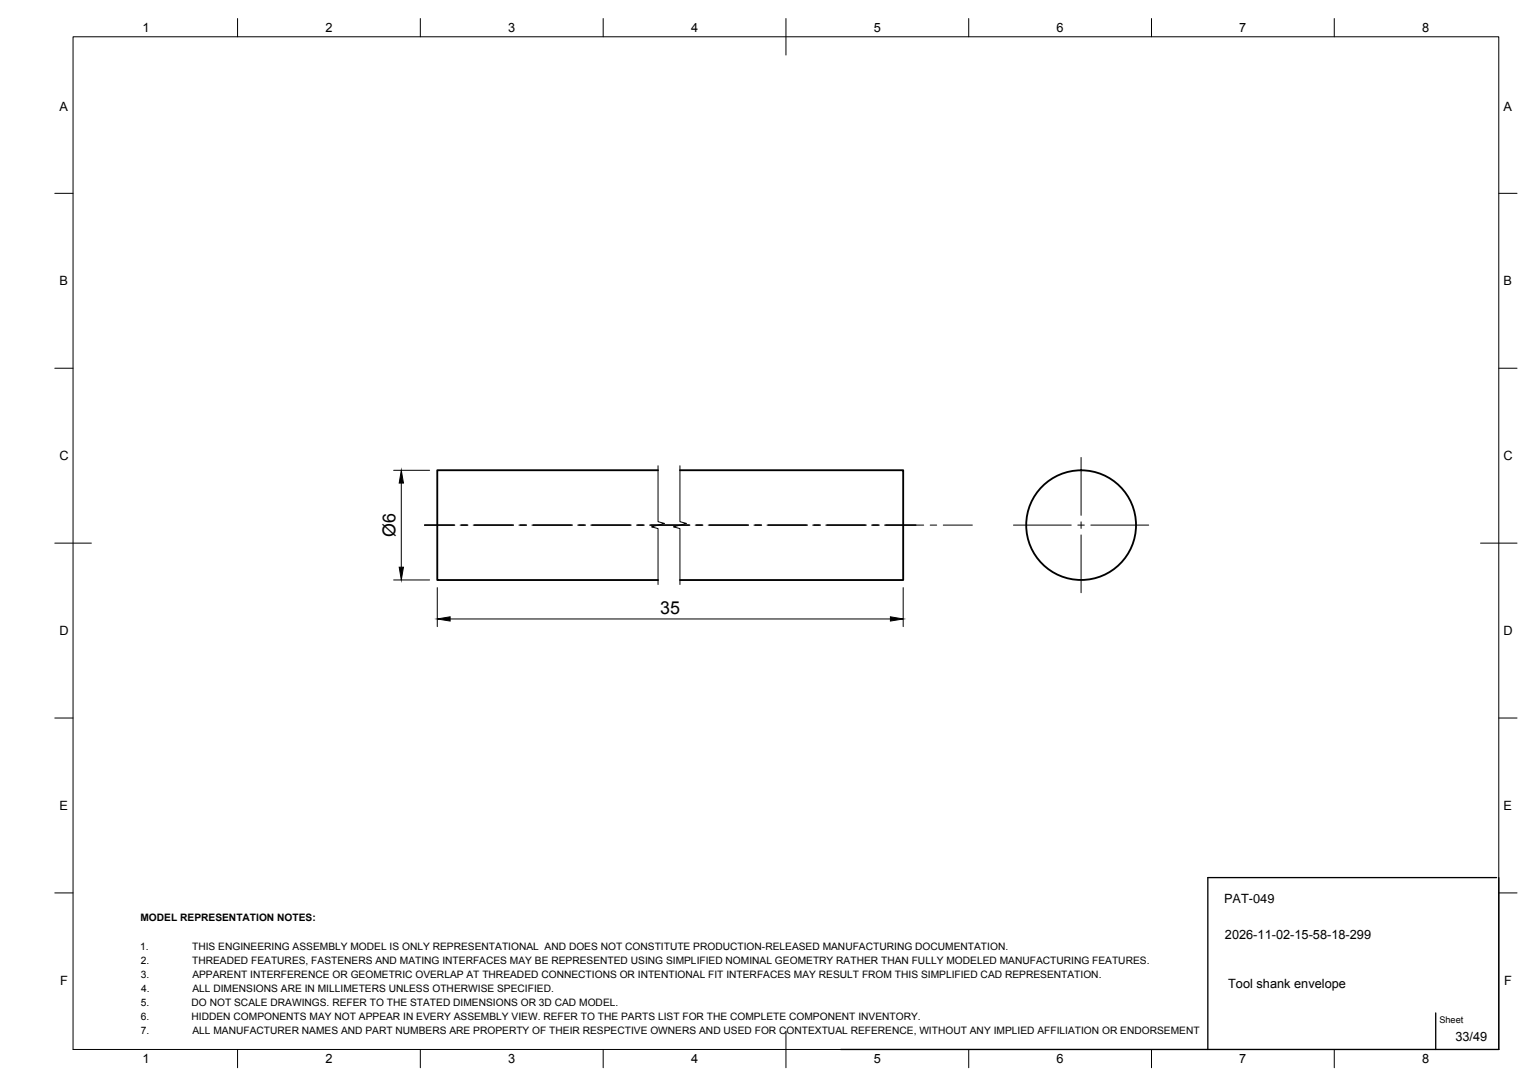
ISO-10303-21;
HEADER;
/* Generated by software containing ST-Developer
 * from STEP Tools, Inc. (www.steptools.com) 
 */

FILE_DESCRIPTION(
/* description */ ('Hand drill press frame (manual)'),
/* implementation_level */ '2;1');

FILE_NAME(
/* name */ 'Tool shank envelope.step',
/* time_stamp */ '2026-10-28T03:25:28-07:00',
/* author */ (''),
/* organization */ (''),
/* preprocessor_version */ 'ST-DEVELOPER v20.2',
/* originating_system */ 'Autodesk Translation Framework v15.17.0.0',
/* authorisation */ '');

FILE_SCHEMA (('AUTOMOTIVE_DESIGN { 1 0 10303 214 3 1 1 }'));
ENDSEC;

DATA;
#10=MECHANICAL_DESIGN_GEOMETRIC_PRESENTATION_REPRESENTATION('',(#651),#33299);
#554=SHAPE_REPRESENTATION_RELATIONSHIP('SRR','None',#33515,#599);
#599=ADVANCED_BREP_SHAPE_REPRESENTATION('',(#702),#33277);
#651=STYLED_ITEM('',(#33807),#702);
#702=MANIFOLD_SOLID_BREP('Body1',#12670);
#1219=PLANE('',#13959);
#1220=PLANE('',#13960);
#1801=FACE_OUTER_BOUND('',#2622,.T.);
#1802=FACE_OUTER_BOUND('',#2623,.T.);
#1803=FACE_OUTER_BOUND('',#2624,.T.);
#2622=EDGE_LOOP('',(#10757,#10758,#10759,#10760));
#2623=EDGE_LOOP('',(#10761));
#2624=EDGE_LOOP('',(#10762));
#3747=LINE('',#20875,#4912);
#4912=VECTOR('',#16770,0.3);
#5485=CIRCLE('',#13957,0.3);
#5486=CIRCLE('',#13958,0.3);
#6399=VERTEX_POINT('',#20872);
#6400=VERTEX_POINT('',#20874);
#7907=EDGE_CURVE('',#6399,#6399,#5485,.T.);
#7908=EDGE_CURVE('',#6399,#6400,#3747,.T.);
#7909=EDGE_CURVE('',#6400,#6400,#5486,.T.);
#10757=ORIENTED_EDGE('',*,*,#7907,.F.);
#10758=ORIENTED_EDGE('',*,*,#7908,.T.);
#10759=ORIENTED_EDGE('',*,*,#7909,.T.);
#10760=ORIENTED_EDGE('',*,*,#7908,.F.);
#10761=ORIENTED_EDGE('',*,*,#7907,.T.);
#10762=ORIENTED_EDGE('',*,*,#7909,.F.);
#11891=CYLINDRICAL_SURFACE('',#13956,0.3);
#12410=ADVANCED_FACE('',(#1801),#11891,.T.);
#12411=ADVANCED_FACE('',(#1802),#1219,.T.);
#12412=ADVANCED_FACE('',(#1803),#1220,.F.);
#12670=CLOSED_SHELL('',(#12410,#12411,#12412));
#13955=AXIS2_PLACEMENT_3D('',#20870,#16764,#16765);
#13956=AXIS2_PLACEMENT_3D('',#20871,#16766,#16767);
#13957=AXIS2_PLACEMENT_3D('',#20873,#16768,#16769);
#13958=AXIS2_PLACEMENT_3D('',#20876,#16771,#16772);
#13959=AXIS2_PLACEMENT_3D('',#20877,#16773,#16774);
#13960=AXIS2_PLACEMENT_3D('',#20878,#16775,#16776);
#16764=DIRECTION('axis',(0.,0.,1.));
#16765=DIRECTION('refdir',(1.,0.,0.));
#16766=DIRECTION('center_axis',(0.,0.,1.));
#16767=DIRECTION('ref_axis',(1.,0.,0.));
#16768=DIRECTION('center_axis',(0.,0.,1.));
#16769=DIRECTION('ref_axis',(1.,0.,0.));
#16770=DIRECTION('',(0.,0.,-1.));
#16771=DIRECTION('center_axis',(0.,0.,1.));
#16772=DIRECTION('ref_axis',(1.,0.,0.));
#16773=DIRECTION('center_axis',(0.,0.,1.));
#16774=DIRECTION('ref_axis',(1.,0.,0.));
#16775=DIRECTION('center_axis',(0.,0.,1.));
#16776=DIRECTION('ref_axis',(1.,0.,0.));
#20870=CARTESIAN_POINT('',(0.,0.,0.));
#20871=CARTESIAN_POINT('Origin',(1.,0.,7.));
#20872=CARTESIAN_POINT('',(0.7,-3.67394039744206E-17,10.5));
#20873=CARTESIAN_POINT('Origin',(1.,0.,10.5));
#20874=CARTESIAN_POINT('',(0.7,-3.67394039744206E-17,7.));
#20875=CARTESIAN_POINT('',(0.7,-3.67394039744206E-17,7.));
#20876=CARTESIAN_POINT('Origin',(1.,0.,7.));
#20877=CARTESIAN_POINT('Origin',(1.,0.,10.5));
#20878=CARTESIAN_POINT('Origin',(1.,0.,7.));
#33225=UNCERTAINTY_MEASURE_WITH_UNIT(LENGTH_MEASURE(0.001),#33300,
'DISTANCE_ACCURACY_VALUE',
'Maximum model space distance between geometric entities at asserted c
onnectivities');
#33247=UNCERTAINTY_MEASURE_WITH_UNIT(LENGTH_MEASURE(0.001),#33300,
'DISTANCE_ACCURACY_VALUE',
'Maximum model space distance between geometric entities at asserted c
onnectivities');
#33277=(
GEOMETRIC_REPRESENTATION_CONTEXT(3)
GLOBAL_UNCERTAINTY_ASSIGNED_CONTEXT((#33225))
GLOBAL_UNIT_ASSIGNED_CONTEXT((#33300,#33302,#33303))
REPRESENTATION_CONTEXT('','3D')
);
#33299=(
GEOMETRIC_REPRESENTATION_CONTEXT(3)
GLOBAL_UNCERTAINTY_ASSIGNED_CONTEXT((#33247))
GLOBAL_UNIT_ASSIGNED_CONTEXT((#33300,#33302,#33303))
REPRESENTATION_CONTEXT('','3D')
);
#33300=(
LENGTH_UNIT()
NAMED_UNIT(*)
SI_UNIT(.CENTI.,.METRE.)
);
#33302=(
NAMED_UNIT(*)
PLANE_ANGLE_UNIT()
SI_UNIT($,.RADIAN.)
);
#33303=(
NAMED_UNIT(*)
SI_UNIT($,.STERADIAN.)
SOLID_ANGLE_UNIT()
);
#33333=SHAPE_DEFINITION_REPRESENTATION(#33389,#33515);
#33389=PRODUCT_DEFINITION_SHAPE('',$,#33567);
#33515=SHAPE_REPRESENTATION('',(#13955),#33277);
#33537=PRODUCT_DEFINITION_CONTEXT('part definition',#33692,'design');
#33567=PRODUCT_DEFINITION('Tool shank envelope','Tool shank envelope',#33618,
#33537);
#33618=PRODUCT_DEFINITION_FORMATION('',$,#33723);
#33692=APPLICATION_CONTEXT(
'Core Data for Automotive Mechanical Design Process');
#33693=PRODUCT_CONTEXT('part definition',#33692,'mechanical');
#33723=PRODUCT('Tool shank envelope','Tool shank envelope',
'Tool shank envelope',(#33693));
#33801=COLOUR_RGB('Sky Blue',0.24,0.69,0.87);
#33802=FILL_AREA_STYLE_COLOUR('',#33801);
#33803=FILL_AREA_STYLE('',(#33802));
#33804=SURFACE_STYLE_FILL_AREA(#33803);
#33805=SURFACE_SIDE_STYLE('',(#33804));
#33806=SURFACE_STYLE_USAGE(.BOTH.,#33805);
#33807=PRESENTATION_STYLE_ASSIGNMENT((#33806));
ENDSEC;
END-ISO-10303-21;
